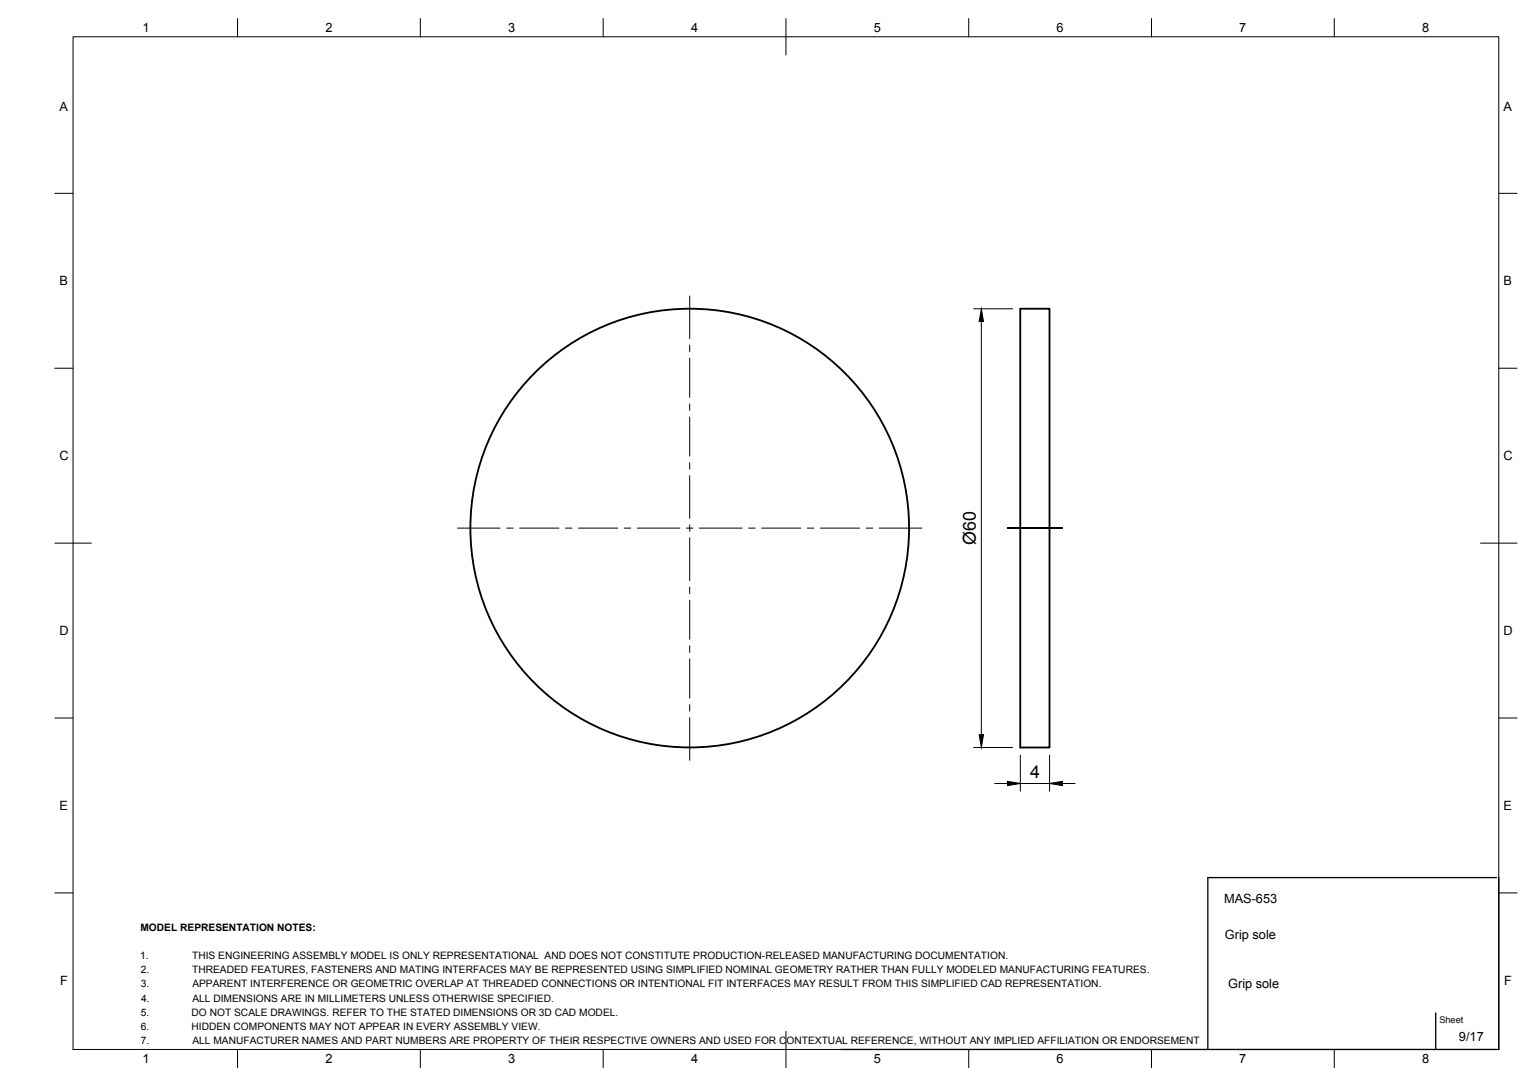
ISO-10303-21;
HEADER;
/* Generated by software containing ST-Developer
 * from STEP Tools, Inc. (www.steptools.com) 
 */

FILE_DESCRIPTION(
/* description */ ('Independent compact industrial fixture table, bolted aluminum worktop
 on connected adjustable support base. Whole-mm nominal dimensions. No
 load rating assigned.'),
/* implementation_level */ '2;1');

FILE_NAME(
/* name */ 'Grip sole.step',
/* time_stamp */ '2026-11-07T17:47:58-08:00',
/* author */ (''),
/* organization */ (''),
/* preprocessor_version */ 'ST-DEVELOPER v20.2',
/* originating_system */ 'Autodesk Translation Framework v15.17.0.0',
/* authorisation */ '');

FILE_SCHEMA (('AUTOMOTIVE_DESIGN { 1 0 10303 214 3 1 1 }'));
ENDSEC;

DATA;
#10=MECHANICAL_DESIGN_GEOMETRIC_PRESENTATION_REPRESENTATION('',(#2258),#97475);
#2220=SHAPE_REPRESENTATION_RELATIONSHIP('SRR','None',#97614,#2239);
#2239=ADVANCED_BREP_SHAPE_REPRESENTATION('',(#2277),#97464);
#2258=STYLED_ITEM('',(#97720),#2277);
#2277=MANIFOLD_SOLID_BREP('Body1',#21819);
#2476=PLANE('',#22699);
#2477=PLANE('',#22700);
#3005=FACE_OUTER_BOUND('',#4212,.T.);
#3006=FACE_OUTER_BOUND('',#4213,.T.);
#3007=FACE_OUTER_BOUND('',#4214,.T.);
#4212=EDGE_LOOP('',(#15782,#15783,#15784,#15785));
#4213=EDGE_LOOP('',(#15786));
#4214=EDGE_LOOP('',(#15787));
#5493=LINE('',#56448,#6707);
#6707=VECTOR('',#25375,30.);
#7516=CIRCLE('',#22697,30.);
#7517=CIRCLE('',#22698,30.);
#8503=VERTEX_POINT('',#56445);
#8504=VERTEX_POINT('',#56447);
#11148=EDGE_CURVE('',#8503,#8503,#7516,.T.);
#11149=EDGE_CURVE('',#8503,#8504,#5493,.T.);
#11150=EDGE_CURVE('',#8504,#8504,#7517,.T.);
#15782=ORIENTED_EDGE('',*,*,#11148,.F.);
#15783=ORIENTED_EDGE('',*,*,#11149,.T.);
#15784=ORIENTED_EDGE('',*,*,#11150,.T.);
#15785=ORIENTED_EDGE('',*,*,#11149,.F.);
#15786=ORIENTED_EDGE('',*,*,#11148,.T.);
#15787=ORIENTED_EDGE('',*,*,#11150,.F.);
#20063=CYLINDRICAL_SURFACE('',#22696,30.);
#21125=ADVANCED_FACE('',(#3005),#20063,.T.);
#21126=ADVANCED_FACE('',(#3006),#2476,.T.);
#21127=ADVANCED_FACE('',(#3007),#2477,.F.);
#21819=CLOSED_SHELL('',(#21125,#21126,#21127));
#22695=AXIS2_PLACEMENT_3D('',#56443,#25369,#25370);
#22696=AXIS2_PLACEMENT_3D('',#56444,#25371,#25372);
#22697=AXIS2_PLACEMENT_3D('',#56446,#25373,#25374);
#22698=AXIS2_PLACEMENT_3D('',#56449,#25376,#25377);
#22699=AXIS2_PLACEMENT_3D('',#56450,#25378,#25379);
#22700=AXIS2_PLACEMENT_3D('',#56451,#25380,#25381);
#25369=DIRECTION('axis',(0.,0.,1.));
#25370=DIRECTION('refdir',(1.,0.,0.));
#25371=DIRECTION('center_axis',(0.,0.,1.));
#25372=DIRECTION('ref_axis',(1.,0.,0.));
#25373=DIRECTION('center_axis',(0.,0.,1.));
#25374=DIRECTION('ref_axis',(1.,0.,0.));
#25375=DIRECTION('',(0.,0.,-1.));
#25376=DIRECTION('center_axis',(0.,0.,1.));
#25377=DIRECTION('ref_axis',(1.,0.,0.));
#25378=DIRECTION('center_axis',(0.,0.,1.));
#25379=DIRECTION('ref_axis',(1.,0.,0.));
#25380=DIRECTION('center_axis',(0.,0.,1.));
#25381=DIRECTION('ref_axis',(1.,0.,0.));
#56443=CARTESIAN_POINT('',(0.,0.,0.));
#56444=CARTESIAN_POINT('Origin',(0.,0.,0.));
#56445=CARTESIAN_POINT('',(-30.,-3.67394039744206E-15,4.));
#56446=CARTESIAN_POINT('Origin',(0.,0.,4.));
#56447=CARTESIAN_POINT('',(-30.,-3.67394039744206E-15,0.));
#56448=CARTESIAN_POINT('',(-30.,-3.67394039744206E-15,0.));
#56449=CARTESIAN_POINT('Origin',(0.,0.,0.));
#56450=CARTESIAN_POINT('Origin',(0.,0.,4.));
#56451=CARTESIAN_POINT('Origin',(0.,0.,0.));
#97441=UNCERTAINTY_MEASURE_WITH_UNIT(LENGTH_MEASURE(0.01),#97476,
'DISTANCE_ACCURACY_VALUE',
'Maximum model space distance between geometric entities at asserted c
onnectivities');
#97452=UNCERTAINTY_MEASURE_WITH_UNIT(LENGTH_MEASURE(0.01),#97476,
'DISTANCE_ACCURACY_VALUE',
'Maximum model space distance between geometric entities at asserted c
onnectivities');
#97464=(
GEOMETRIC_REPRESENTATION_CONTEXT(3)
GLOBAL_UNCERTAINTY_ASSIGNED_CONTEXT((#97441))
GLOBAL_UNIT_ASSIGNED_CONTEXT((#97476,#97478,#97479))
REPRESENTATION_CONTEXT('','3D')
);
#97475=(
GEOMETRIC_REPRESENTATION_CONTEXT(3)
GLOBAL_UNCERTAINTY_ASSIGNED_CONTEXT((#97452))
GLOBAL_UNIT_ASSIGNED_CONTEXT((#97476,#97478,#97479))
REPRESENTATION_CONTEXT('','3D')
);
#97476=(
LENGTH_UNIT()
NAMED_UNIT(*)
SI_UNIT(.MILLI.,.METRE.)
);
#97478=(
NAMED_UNIT(*)
PLANE_ANGLE_UNIT()
SI_UNIT($,.RADIAN.)
);
#97479=(
NAMED_UNIT(*)
SI_UNIT($,.STERADIAN.)
SOLID_ANGLE_UNIT()
);
#97491=SHAPE_DEFINITION_REPRESENTATION(#97553,#97614);
#97553=PRODUCT_DEFINITION_SHAPE('',$,#97637);
#97614=SHAPE_REPRESENTATION('',(#22695),#97464);
#97625=PRODUCT_DEFINITION_CONTEXT('part definition',#97693,'design');
#97637=PRODUCT_DEFINITION('Grip sole','Grip sole',#97659,#97625);
#97659=PRODUCT_DEFINITION_FORMATION('',$,#97706);
#97693=APPLICATION_CONTEXT(
'Core Data for Automotive Mechanical Design Process');
#97694=PRODUCT_CONTEXT('part definition',#97693,'mechanical');
#97706=PRODUCT('Grip sole','Grip sole',
'Bonded elastomer sole; nominal diameter 60 mm, thickness 4 mm.',(#97694));
#97720=PRESENTATION_STYLE_ASSIGNMENT((#97727));
#97727=SURFACE_STYLE_USAGE(.BOTH.,#97734);
#97734=SURFACE_SIDE_STYLE('',(#97741));
#97741=SURFACE_STYLE_FILL_AREA(#97748);
#97748=FILL_AREA_STYLE('Dark gray',(#97755));
#97755=FILL_AREA_STYLE_COLOUR('Dark gray',#97762);
#97762=COLOUR_RGB('Dark gray',0.250980392156863,0.282352941176471,0.32156862745098);
ENDSEC;
END-ISO-10303-21;
